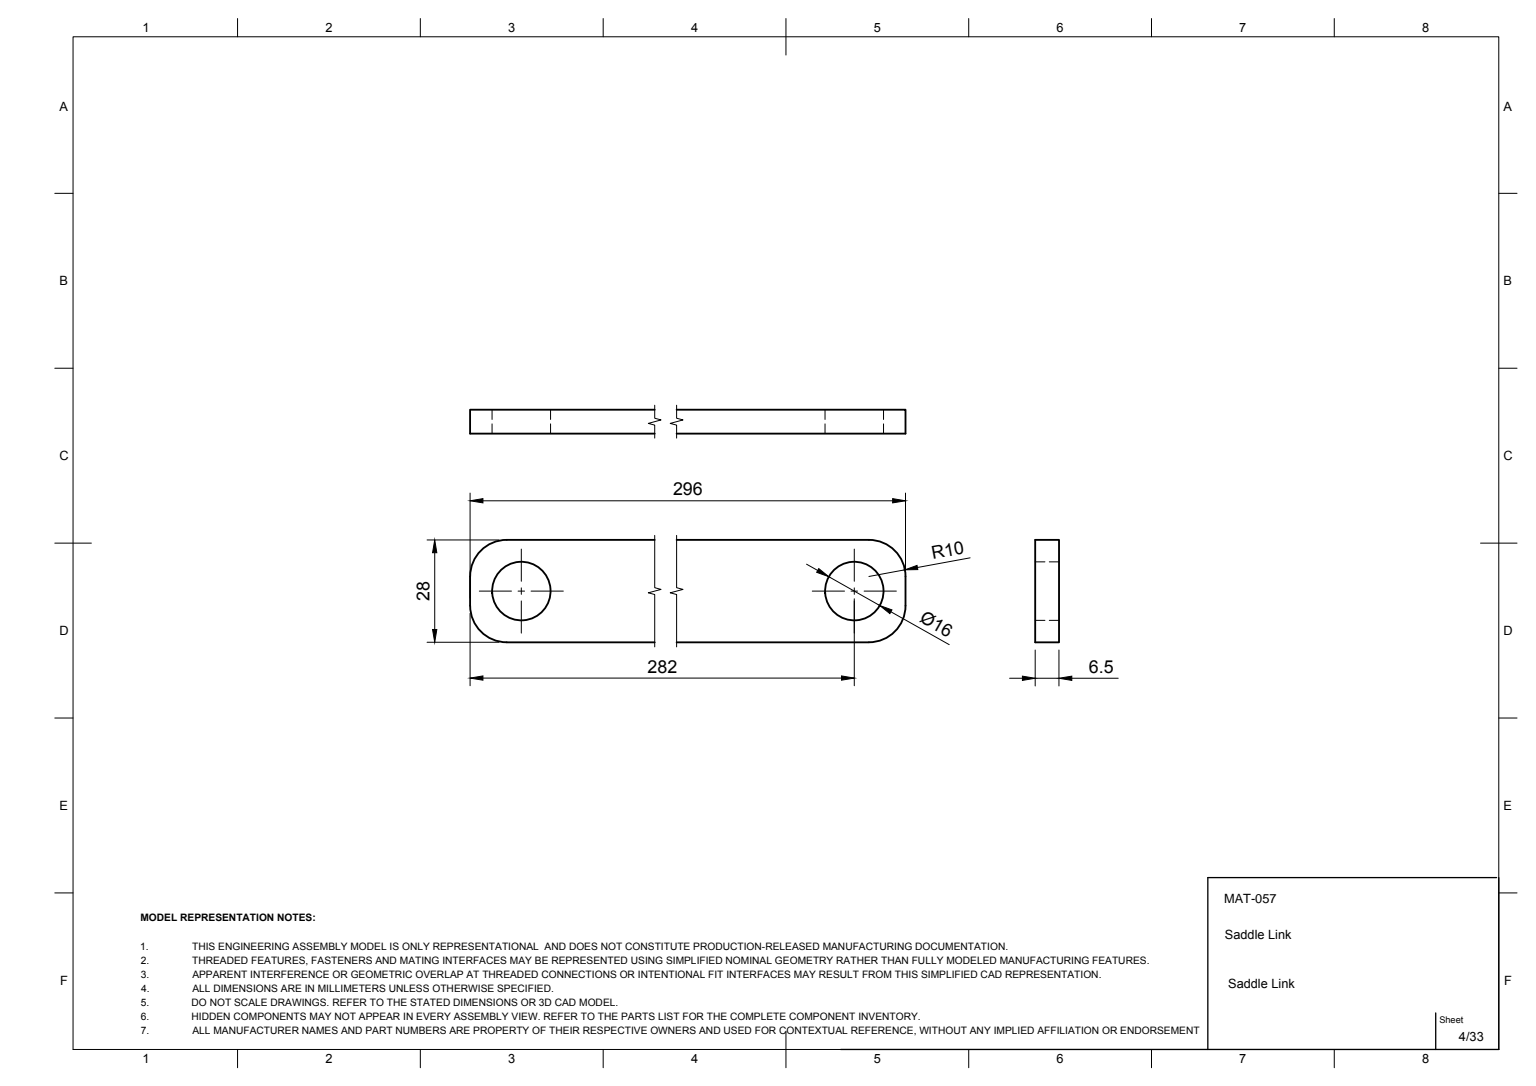
ISO-10303-21;
HEADER;
/* Generated by software containing ST-Developer
 * from STEP Tools, Inc. (www.steptools.com) 
 */

FILE_DESCRIPTION(
/* description */ ('STEP AP214', 'CAx-IF Rec.Pracs.---Representation and Presentation of Product Manufa
cturing Information (PMI)---4.0---2014-10-13'),
/* implementation_level */ '2;1');

FILE_NAME(
/* name */ 'Saddle Link.step',
/* time_stamp */ '2026-10-28T23:34:22+01:00',
/* author */ (''),
/* organization */ (''),
/* preprocessor_version */ 'ST-DEVELOPER v20.2',
/* originating_system */ 'Autodesk Translation Framework v15.17.0.0',
/* authorisation */ '');

FILE_SCHEMA (('AP242_MANAGED_MODEL_BASED_3D_ENGINEERING_MIM_LF { 1 0 10303 442 2 1 4 }'));
ENDSEC;

DATA;
#10=MECHANICAL_DESIGN_GEOMETRIC_PRESENTATION_REPRESENTATION('',(#258),#27807);
#212=SHAPE_REPRESENTATION_RELATIONSHIP('SRR','None',#27908,#234);
#234=ADVANCED_BREP_SHAPE_REPRESENTATION('',(#287),#27788);
#258=STYLED_ITEM('',(#28091),#287);
#287=MANIFOLD_SOLID_BREP('Body1',#12034);
#393=FACE_BOUND('',#2309,.T.);
#394=FACE_BOUND('',#2310,.T.);
#395=FACE_BOUND('',#2312,.T.);
#396=FACE_BOUND('',#2313,.T.);
#582=PLANE('',#12975);
#583=PLANE('',#12980);
#584=PLANE('',#12985);
#585=PLANE('',#12986);
#586=PLANE('',#12987);
#587=PLANE('',#12988);
#1093=CYLINDRICAL_SURFACE('',#12969,8.00000000000002);
#1094=CYLINDRICAL_SURFACE('',#12972,8.00000000000001);
#1095=CYLINDRICAL_SURFACE('',#12989,10.);
#1096=CYLINDRICAL_SURFACE('',#12990,9.99999999999999);
#1097=CYLINDRICAL_SURFACE('',#12991,10.);
#1098=CYLINDRICAL_SURFACE('',#12992,10.);
#1551=FACE_OUTER_BOUND('',#2306,.T.);
#1552=FACE_OUTER_BOUND('',#2307,.T.);
#1553=FACE_OUTER_BOUND('',#2308,.T.);
#1554=FACE_OUTER_BOUND('',#2311,.T.);
#1555=FACE_OUTER_BOUND('',#2314,.T.);
#1556=FACE_OUTER_BOUND('',#2315,.T.);
#1557=FACE_OUTER_BOUND('',#2316,.T.);
#1558=FACE_OUTER_BOUND('',#2317,.T.);
#1559=FACE_OUTER_BOUND('',#2318,.T.);
#1560=FACE_OUTER_BOUND('',#2319,.T.);
#1561=FACE_OUTER_BOUND('',#2320,.T.);
#1562=FACE_OUTER_BOUND('',#2321,.T.);
#2306=EDGE_LOOP('',(#9421,#9422,#9423,#9424));
#2307=EDGE_LOOP('',(#9425,#9426,#9427,#9428));
#2308=EDGE_LOOP('',(#9429,#9430,#9431,#9432,#9433,#9434,#9435,#9436));
#2309=EDGE_LOOP('',(#9437));
#2310=EDGE_LOOP('',(#9438));
#2311=EDGE_LOOP('',(#9439,#9440,#9441,#9442,#9443,#9444,#9445,#9446));
#2312=EDGE_LOOP('',(#9447));
#2313=EDGE_LOOP('',(#9448));
#2314=EDGE_LOOP('',(#9449,#9450,#9451,#9452));
#2315=EDGE_LOOP('',(#9453,#9454,#9455,#9456));
#2316=EDGE_LOOP('',(#9457,#9458,#9459,#9460));
#2317=EDGE_LOOP('',(#9461,#9462,#9463,#9464));
#2318=EDGE_LOOP('',(#9465,#9466,#9467,#9468));
#2319=EDGE_LOOP('',(#9469,#9470,#9471,#9472));
#2320=EDGE_LOOP('',(#9473,#9474,#9475,#9476));
#2321=EDGE_LOOP('',(#9477,#9478,#9479,#9480));
#3142=LINE('',#19340,#3962);
#3143=LINE('',#19346,#3963);
#3144=LINE('',#19351,#3964);
#3145=LINE('',#19355,#3965);
#3146=LINE('',#19359,#3966);
#3147=LINE('',#19363,#3967);
#3148=LINE('',#19368,#3968);
#3149=LINE('',#19372,#3969);
#3150=LINE('',#19376,#3970);
#3151=LINE('',#19380,#3971);
#3152=LINE('',#19383,#3972);
#3153=LINE('',#19384,#3973);
#3154=LINE('',#19386,#3974);
#3155=LINE('',#19387,#3975);
#3156=LINE('',#19389,#3976);
#3157=LINE('',#19390,#3977);
#3158=LINE('',#19392,#3978);
#3159=LINE('',#19393,#3979);
#3962=VECTOR('',#15466,8.00000000000002);
#3963=VECTOR('',#15473,8.00000000000001);
#3964=VECTOR('',#15478,1000.);
#3965=VECTOR('',#15481,1000.);
#3966=VECTOR('',#15484,1000.);
#3967=VECTOR('',#15487,1000.);
#3968=VECTOR('',#15492,1000.);
#3969=VECTOR('',#15495,1000.);
#3970=VECTOR('',#15498,1000.);
#3971=VECTOR('',#15501,1000.);
#3972=VECTOR('',#15506,1000.);
#3973=VECTOR('',#15507,1000.);
#3974=VECTOR('',#15510,1000.);
#3975=VECTOR('',#15511,1000.);
#3976=VECTOR('',#15514,1000.);
#3977=VECTOR('',#15515,1000.);
#3978=VECTOR('',#15518,1000.);
#3979=VECTOR('',#15519,1000.);
#4723=CIRCLE('',#12970,7.99999999999999);
#4724=CIRCLE('',#12971,7.99999999999999);
#4725=CIRCLE('',#12973,8.00000000000001);
#4726=CIRCLE('',#12974,8.00000000000001);
#4727=CIRCLE('',#12976,10.);
#4728=CIRCLE('',#12977,10.);
#4729=CIRCLE('',#12978,10.);
#4730=CIRCLE('',#12979,10.);
#4731=CIRCLE('',#12981,10.);
#4732=CIRCLE('',#12982,10.);
#4733=CIRCLE('',#12983,10.);
#4734=CIRCLE('',#12984,10.);
#5544=VERTEX_POINT('',#19337);
#5545=VERTEX_POINT('',#19339);
#5546=VERTEX_POINT('',#19343);
#5547=VERTEX_POINT('',#19345);
#5548=VERTEX_POINT('',#19349);
#5549=VERTEX_POINT('',#19350);
#5550=VERTEX_POINT('',#19352);
#5551=VERTEX_POINT('',#19354);
#5552=VERTEX_POINT('',#19356);
#5553=VERTEX_POINT('',#19358);
#5554=VERTEX_POINT('',#19360);
#5555=VERTEX_POINT('',#19362);
#5556=VERTEX_POINT('',#19366);
#5557=VERTEX_POINT('',#19367);
#5558=VERTEX_POINT('',#19369);
#5559=VERTEX_POINT('',#19371);
#5560=VERTEX_POINT('',#19373);
#5561=VERTEX_POINT('',#19375);
#5562=VERTEX_POINT('',#19377);
#5563=VERTEX_POINT('',#19379);
#6923=EDGE_CURVE('',#5544,#5544,#4723,.T.);
#6924=EDGE_CURVE('',#5544,#5545,#3142,.T.);
#6925=EDGE_CURVE('',#5545,#5545,#4724,.T.);
#6926=EDGE_CURVE('',#5546,#5546,#4725,.T.);
#6927=EDGE_CURVE('',#5546,#5547,#3143,.T.);
#6928=EDGE_CURVE('',#5547,#5547,#4726,.T.);
#6929=EDGE_CURVE('',#5548,#5549,#3144,.T.);
#6930=EDGE_CURVE('',#5549,#5550,#4727,.T.);
#6931=EDGE_CURVE('',#5550,#5551,#3145,.T.);
#6932=EDGE_CURVE('',#5551,#5552,#4728,.T.);
#6933=EDGE_CURVE('',#5552,#5553,#3146,.T.);
#6934=EDGE_CURVE('',#5553,#5554,#4729,.T.);
#6935=EDGE_CURVE('',#5554,#5555,#3147,.T.);
#6936=EDGE_CURVE('',#5555,#5548,#4730,.T.);
#6937=EDGE_CURVE('',#5556,#5557,#3148,.T.);
#6938=EDGE_CURVE('',#5556,#5558,#4731,.T.);
#6939=EDGE_CURVE('',#5559,#5558,#3149,.T.);
#6940=EDGE_CURVE('',#5559,#5560,#4732,.T.);
#6941=EDGE_CURVE('',#5561,#5560,#3150,.T.);
#6942=EDGE_CURVE('',#5561,#5562,#4733,.T.);
#6943=EDGE_CURVE('',#5563,#5562,#3151,.T.);
#6944=EDGE_CURVE('',#5563,#5557,#4734,.T.);
#6945=EDGE_CURVE('',#5550,#5556,#3152,.T.);
#6946=EDGE_CURVE('',#5557,#5551,#3153,.T.);
#6947=EDGE_CURVE('',#5552,#5563,#3154,.T.);
#6948=EDGE_CURVE('',#5562,#5553,#3155,.T.);
#6949=EDGE_CURVE('',#5560,#5555,#3156,.T.);
#6950=EDGE_CURVE('',#5554,#5561,#3157,.T.);
#6951=EDGE_CURVE('',#5558,#5549,#3158,.T.);
#6952=EDGE_CURVE('',#5548,#5559,#3159,.T.);
#9421=ORIENTED_EDGE('',*,*,#6923,.T.);
#9422=ORIENTED_EDGE('',*,*,#6924,.T.);
#9423=ORIENTED_EDGE('',*,*,#6925,.F.);
#9424=ORIENTED_EDGE('',*,*,#6924,.F.);
#9425=ORIENTED_EDGE('',*,*,#6926,.T.);
#9426=ORIENTED_EDGE('',*,*,#6927,.T.);
#9427=ORIENTED_EDGE('',*,*,#6928,.F.);
#9428=ORIENTED_EDGE('',*,*,#6927,.F.);
#9429=ORIENTED_EDGE('',*,*,#6929,.T.);
#9430=ORIENTED_EDGE('',*,*,#6930,.T.);
#9431=ORIENTED_EDGE('',*,*,#6931,.T.);
#9432=ORIENTED_EDGE('',*,*,#6932,.T.);
#9433=ORIENTED_EDGE('',*,*,#6933,.T.);
#9434=ORIENTED_EDGE('',*,*,#6934,.T.);
#9435=ORIENTED_EDGE('',*,*,#6935,.T.);
#9436=ORIENTED_EDGE('',*,*,#6936,.T.);
#9437=ORIENTED_EDGE('',*,*,#6923,.F.);
#9438=ORIENTED_EDGE('',*,*,#6926,.F.);
#9439=ORIENTED_EDGE('',*,*,#6937,.F.);
#9440=ORIENTED_EDGE('',*,*,#6938,.T.);
#9441=ORIENTED_EDGE('',*,*,#6939,.F.);
#9442=ORIENTED_EDGE('',*,*,#6940,.T.);
#9443=ORIENTED_EDGE('',*,*,#6941,.F.);
#9444=ORIENTED_EDGE('',*,*,#6942,.T.);
#9445=ORIENTED_EDGE('',*,*,#6943,.F.);
#9446=ORIENTED_EDGE('',*,*,#6944,.T.);
#9447=ORIENTED_EDGE('',*,*,#6928,.T.);
#9448=ORIENTED_EDGE('',*,*,#6925,.T.);
#9449=ORIENTED_EDGE('',*,*,#6931,.F.);
#9450=ORIENTED_EDGE('',*,*,#6945,.T.);
#9451=ORIENTED_EDGE('',*,*,#6937,.T.);
#9452=ORIENTED_EDGE('',*,*,#6946,.T.);
#9453=ORIENTED_EDGE('',*,*,#6933,.F.);
#9454=ORIENTED_EDGE('',*,*,#6947,.T.);
#9455=ORIENTED_EDGE('',*,*,#6943,.T.);
#9456=ORIENTED_EDGE('',*,*,#6948,.T.);
#9457=ORIENTED_EDGE('',*,*,#6941,.T.);
#9458=ORIENTED_EDGE('',*,*,#6949,.T.);
#9459=ORIENTED_EDGE('',*,*,#6935,.F.);
#9460=ORIENTED_EDGE('',*,*,#6950,.T.);
#9461=ORIENTED_EDGE('',*,*,#6939,.T.);
#9462=ORIENTED_EDGE('',*,*,#6951,.T.);
#9463=ORIENTED_EDGE('',*,*,#6929,.F.);
#9464=ORIENTED_EDGE('',*,*,#6952,.T.);
#9465=ORIENTED_EDGE('',*,*,#6930,.F.);
#9466=ORIENTED_EDGE('',*,*,#6951,.F.);
#9467=ORIENTED_EDGE('',*,*,#6938,.F.);
#9468=ORIENTED_EDGE('',*,*,#6945,.F.);
#9469=ORIENTED_EDGE('',*,*,#6932,.F.);
#9470=ORIENTED_EDGE('',*,*,#6946,.F.);
#9471=ORIENTED_EDGE('',*,*,#6944,.F.);
#9472=ORIENTED_EDGE('',*,*,#6947,.F.);
#9473=ORIENTED_EDGE('',*,*,#6936,.F.);
#9474=ORIENTED_EDGE('',*,*,#6949,.F.);
#9475=ORIENTED_EDGE('',*,*,#6940,.F.);
#9476=ORIENTED_EDGE('',*,*,#6952,.F.);
#9477=ORIENTED_EDGE('',*,*,#6934,.F.);
#9478=ORIENTED_EDGE('',*,*,#6948,.F.);
#9479=ORIENTED_EDGE('',*,*,#6942,.F.);
#9480=ORIENTED_EDGE('',*,*,#6950,.F.);
#11633=ADVANCED_FACE('',(#1551),#1093,.F.);
#11634=ADVANCED_FACE('',(#1552),#1094,.F.);
#11635=ADVANCED_FACE('',(#1553,#393,#394),#582,.T.);
#11636=ADVANCED_FACE('',(#1554,#395,#396),#583,.F.);
#11637=ADVANCED_FACE('',(#1555),#584,.F.);
#11638=ADVANCED_FACE('',(#1556),#585,.F.);
#11639=ADVANCED_FACE('',(#1557),#586,.F.);
#11640=ADVANCED_FACE('',(#1558),#587,.F.);
#11641=ADVANCED_FACE('',(#1559),#1095,.T.);
#11642=ADVANCED_FACE('',(#1560),#1096,.T.);
#11643=ADVANCED_FACE('',(#1561),#1097,.T.);
#11644=ADVANCED_FACE('',(#1562),#1098,.T.);
#12034=CLOSED_SHELL('',(#11633,#11634,#11635,#11636,#11637,#11638,#11639,
#11640,#11641,#11642,#11643,#11644));
#12968=AXIS2_PLACEMENT_3D('',#19335,#15460,#15461);
#12969=AXIS2_PLACEMENT_3D('',#19336,#15462,#15463);
#12970=AXIS2_PLACEMENT_3D('',#19338,#15464,#15465);
#12971=AXIS2_PLACEMENT_3D('',#19341,#15467,#15468);
#12972=AXIS2_PLACEMENT_3D('',#19342,#15469,#15470);
#12973=AXIS2_PLACEMENT_3D('',#19344,#15471,#15472);
#12974=AXIS2_PLACEMENT_3D('',#19347,#15474,#15475);
#12975=AXIS2_PLACEMENT_3D('',#19348,#15476,#15477);
#12976=AXIS2_PLACEMENT_3D('',#19353,#15479,#15480);
#12977=AXIS2_PLACEMENT_3D('',#19357,#15482,#15483);
#12978=AXIS2_PLACEMENT_3D('',#19361,#15485,#15486);
#12979=AXIS2_PLACEMENT_3D('',#19364,#15488,#15489);
#12980=AXIS2_PLACEMENT_3D('',#19365,#15490,#15491);
#12981=AXIS2_PLACEMENT_3D('',#19370,#15493,#15494);
#12982=AXIS2_PLACEMENT_3D('',#19374,#15496,#15497);
#12983=AXIS2_PLACEMENT_3D('',#19378,#15499,#15500);
#12984=AXIS2_PLACEMENT_3D('',#19381,#15502,#15503);
#12985=AXIS2_PLACEMENT_3D('',#19382,#15504,#15505);
#12986=AXIS2_PLACEMENT_3D('',#19385,#15508,#15509);
#12987=AXIS2_PLACEMENT_3D('',#19388,#15512,#15513);
#12988=AXIS2_PLACEMENT_3D('',#19391,#15516,#15517);
#12989=AXIS2_PLACEMENT_3D('',#19394,#15520,#15521);
#12990=AXIS2_PLACEMENT_3D('',#19395,#15522,#15523);
#12991=AXIS2_PLACEMENT_3D('',#19396,#15524,#15525);
#12992=AXIS2_PLACEMENT_3D('',#19397,#15526,#15527);
#15460=DIRECTION('axis',(0.,0.,1.));
#15461=DIRECTION('refdir',(1.,0.,0.));
#15462=DIRECTION('center_axis',(1.34374111916937E-16,-6.5016645363134E-17,
1.));
#15463=DIRECTION('ref_axis',(0.997400584683992,-0.0720560453538152,-1.38709660139384E-16));
#15464=DIRECTION('center_axis',(-1.34374111916937E-16,6.5016645363134E-17,
-1.));
#15465=DIRECTION('ref_axis',(-0.997400584683992,0.0720560453538154,1.38709660139384E-16));
#15466=DIRECTION('',(1.34374111916937E-16,-6.5016645363134E-17,1.));
#15467=DIRECTION('center_axis',(-1.34374111916937E-16,6.5016645363134E-17,
-1.));
#15468=DIRECTION('ref_axis',(-0.997400584683992,0.0720560453538154,1.38709660139384E-16));
#15469=DIRECTION('center_axis',(1.34374111916937E-16,-6.5016645363134E-17,
1.));
#15470=DIRECTION('ref_axis',(0.997400584683992,-0.0720560453538153,-1.38709660139384E-16));
#15471=DIRECTION('center_axis',(-1.34374111916937E-16,6.5016645363134E-17,
-1.));
#15472=DIRECTION('ref_axis',(-0.997400584683992,0.0720560453538153,1.38709660139384E-16));
#15473=DIRECTION('',(1.34374111916937E-16,-6.5016645363134E-17,1.));
#15474=DIRECTION('center_axis',(-1.34374111916937E-16,6.5016645363134E-17,
-1.));
#15475=DIRECTION('ref_axis',(-0.997400584683992,0.0720560453538153,1.38709660139384E-16));
#15476=DIRECTION('center_axis',(-9.47320768979473E-17,6.21527526432887E-17,
-1.));
#15477=DIRECTION('ref_axis',(-0.997400584683992,0.072056045353816,9.89643104496708E-17));
#15478=DIRECTION('',(-0.997400584683992,0.072056045353816,9.89643104496708E-17));
#15479=DIRECTION('center_axis',(-1.34374111916937E-16,6.5016645363134E-17,
-1.));
#15480=DIRECTION('ref_axis',(-0.997400584683992,0.0720560453538159,1.38709660139384E-16));
#15481=DIRECTION('',(0.0720560453538158,0.997400584683992,6.43240143985008E-17));
#15482=DIRECTION('center_axis',(-1.34374111916937E-16,6.5016645363134E-17,
-1.));
#15483=DIRECTION('ref_axis',(-0.997400584683992,0.0720560453538159,1.38709660139384E-16));
#15484=DIRECTION('',(0.997400584683992,-0.072056045353816,-9.89643104496708E-17));
#15485=DIRECTION('center_axis',(-1.34374111916937E-16,6.5016645363134E-17,
-1.));
#15486=DIRECTION('ref_axis',(-0.997400584683992,0.072056045353816,1.38709660139384E-16));
#15487=DIRECTION('',(-0.0720560453538158,-0.997400584683992,-6.43240143985008E-17));
#15488=DIRECTION('center_axis',(-1.34374111916937E-16,6.5016645363134E-17,
-1.));
#15489=DIRECTION('ref_axis',(-0.997400584683992,0.072056045353816,1.38709660139384E-16));
#15490=DIRECTION('center_axis',(-9.47320768979473E-17,6.21527526432887E-17,
-1.));
#15491=DIRECTION('ref_axis',(-0.997400584683992,0.072056045353816,9.89643104496708E-17));
#15492=DIRECTION('',(0.0720560453538158,0.997400584683992,6.43240143985008E-17));
#15493=DIRECTION('center_axis',(1.34374111916937E-16,-6.5016645363134E-17,
1.));
#15494=DIRECTION('ref_axis',(-0.997400584683992,0.0720560453538159,1.38709660139384E-16));
#15495=DIRECTION('',(-0.997400584683992,0.072056045353816,9.89643104496708E-17));
#15496=DIRECTION('center_axis',(1.34374111916937E-16,-6.5016645363134E-17,
1.));
#15497=DIRECTION('ref_axis',(-0.997400584683992,0.0720560453538174,1.38709660139384E-16));
#15498=DIRECTION('',(-0.0720560453538158,-0.997400584683992,-6.43240143985008E-17));
#15499=DIRECTION('center_axis',(1.34374111916937E-16,-6.5016645363134E-17,
1.));
#15500=DIRECTION('ref_axis',(-0.997400584683992,0.072056045353816,1.38709660139384E-16));
#15501=DIRECTION('',(0.997400584683992,-0.072056045353816,-9.89643104496708E-17));
#15502=DIRECTION('center_axis',(1.34374111916937E-16,-6.5016645363134E-17,
1.));
#15503=DIRECTION('ref_axis',(-0.997400584683992,0.0720560453538076,1.38709660139383E-16));
#15504=DIRECTION('center_axis',(0.997400584683992,-0.0720560453538159,-1.38709660139384E-16));
#15505=DIRECTION('ref_axis',(-1.34374111916937E-16,6.5016645363134E-17,
-1.));
#15506=DIRECTION('',(1.34374111916937E-16,-6.5016645363134E-17,1.));
#15507=DIRECTION('',(-1.34374111916937E-16,6.5016645363134E-17,-1.));
#15508=DIRECTION('center_axis',(-0.0720560453538158,-0.997400584683992,
-5.51651729967161E-17));
#15509=DIRECTION('ref_axis',(1.34374111916937E-16,-6.5016645363134E-17,
1.));
#15510=DIRECTION('',(1.34374111916937E-16,-6.5016645363134E-17,1.));
#15511=DIRECTION('',(-1.34374111916937E-16,6.5016645363134E-17,-1.));
#15512=DIRECTION('center_axis',(-0.997400584683992,0.0720560453538159,1.38709660139384E-16));
#15513=DIRECTION('ref_axis',(1.34374111916937E-16,-6.5016645363134E-17,
1.));
#15514=DIRECTION('',(-1.34374111916937E-16,6.5016645363134E-17,-1.));
#15515=DIRECTION('',(1.34374111916937E-16,-6.5016645363134E-17,1.));
#15516=DIRECTION('center_axis',(0.0720560453538158,0.997400584683992,5.51651729967161E-17));
#15517=DIRECTION('ref_axis',(-1.34374111916937E-16,6.5016645363134E-17,
-1.));
#15518=DIRECTION('',(-1.34374111916937E-16,6.5016645363134E-17,-1.));
#15519=DIRECTION('',(1.34374111916937E-16,-6.5016645363134E-17,1.));
#15520=DIRECTION('center_axis',(1.34374111916937E-16,-6.5016645363134E-17,
1.));
#15521=DIRECTION('ref_axis',(0.997400584683992,-0.0720560453538159,-1.38709660139384E-16));
#15522=DIRECTION('center_axis',(1.34374111916937E-16,-6.5016645363134E-17,
1.));
#15523=DIRECTION('ref_axis',(0.997400584683992,-0.0720560453538161,-1.38709660139384E-16));
#15524=DIRECTION('center_axis',(1.34374111916937E-16,-6.5016645363134E-17,
1.));
#15525=DIRECTION('ref_axis',(0.997400584683992,-0.072056045353816,-1.38709660139384E-16));
#15526=DIRECTION('center_axis',(1.34374111916937E-16,-6.5016645363134E-17,
1.));
#15527=DIRECTION('ref_axis',(0.997400584683992,-0.072056045353816,-1.38709660139384E-16));
#19335=CARTESIAN_POINT('',(0.,0.,0.));
#19336=CARTESIAN_POINT('Origin',(-256.262104047423,132.050757761858,278.073593133703));
#19337=CARTESIAN_POINT('',(-264.241308724895,132.627206124688,278.073593133703));
#19338=CARTESIAN_POINT('Origin',(-256.262104047423,132.050757761858,278.073593133703));
#19339=CARTESIAN_POINT('',(-264.241308724895,132.627206124688,284.573593133703));
#19340=CARTESIAN_POINT('',(-264.241308724895,132.627206124688,278.073593133703));
#19341=CARTESIAN_POINT('Origin',(-256.262104047423,132.050757761858,284.573593133703));
#19342=CARTESIAN_POINT('Origin',(11.0412526478865,112.739737607035,278.073593133703));
#19343=CARTESIAN_POINT('',(3.06204797041458,113.316185969866,278.073593133703));
#19344=CARTESIAN_POINT('Origin',(11.0412526478865,112.739737607035,278.073593133703));
#19345=CARTESIAN_POINT('',(3.06204797041458,113.316185969866,284.573593133703));
#19346=CARTESIAN_POINT('',(3.06204797041458,113.316185969866,278.073593133703));
#19347=CARTESIAN_POINT('Origin',(11.0412526478865,112.739737607035,284.573593133703));
#19348=CARTESIAN_POINT('Origin',(-122.610425699768,122.395247684447,278.073593133703));
#19349=CARTESIAN_POINT('',(14.022070351669,98.487905240044,278.073593133703));
#19350=CARTESIAN_POINT('',(-261.260491021113,118.375373757697,278.073593133703));
#19351=CARTESIAN_POINT('',(23.9960761985089,97.7673447865059,278.073593133703));
#19352=CARTESIAN_POINT('',(-270.513936414414,129.069940058075,278.073593133703));
#19353=CARTESIAN_POINT('Origin',(-260.539930567575,128.349379604537,278.073593133703));
#19354=CARTESIAN_POINT('',(-269.937488051584,137.049144735547,278.073593133703));
#19355=CARTESIAN_POINT('',(-269.216927598046,147.023150582387,278.073593133703));
#19356=CARTESIAN_POINT('',(-259.242921751206,146.302590128849,278.073593133703));
#19357=CARTESIAN_POINT('Origin',(-259.963482204744,136.328584282009,278.073593133703));
#19358=CARTESIAN_POINT('',(16.0396396215758,126.415121611196,278.073593133703));
#19359=CARTESIAN_POINT('',(26.0136454684158,125.694561157658,278.073593133703));
#19360=CARTESIAN_POINT('',(25.2930850148776,115.720555310818,278.073593133703));
#19361=CARTESIAN_POINT('Origin',(15.3190791680377,116.441115764356,278.073593133703));
#19362=CARTESIAN_POINT('',(24.7166366520471,107.741350633346,278.073593133703));
#19363=CARTESIAN_POINT('',(26.0136454684158,125.694561157658,278.073593133703));
#19364=CARTESIAN_POINT('Origin',(14.7426308052072,108.461911086884,278.073593133703));
#19365=CARTESIAN_POINT('Origin',(-122.610425699768,122.395247684447,284.573593133703));
#19366=CARTESIAN_POINT('',(-270.513936414414,129.069940058075,284.573593133703));
#19367=CARTESIAN_POINT('',(-269.937488051584,137.049144735547,284.573593133703));
#19368=CARTESIAN_POINT('',(-269.216927598046,147.023150582387,284.573593133703));
#19369=CARTESIAN_POINT('',(-261.260491021113,118.375373757697,284.573593133703));
#19370=CARTESIAN_POINT('Origin',(-260.539930567575,128.349379604537,284.573593133703));
#19371=CARTESIAN_POINT('',(14.022070351669,98.487905240044,284.573593133703));
#19372=CARTESIAN_POINT('',(23.9960761985089,97.7673447865059,284.573593133703));
#19373=CARTESIAN_POINT('',(24.7166366520471,107.741350633346,284.573593133703));
#19374=CARTESIAN_POINT('Origin',(14.7426308052072,108.461911086884,284.573593133703));
#19375=CARTESIAN_POINT('',(25.2930850148776,115.720555310818,284.573593133703));
#19376=CARTESIAN_POINT('',(26.0136454684158,125.694561157658,284.573593133703));
#19377=CARTESIAN_POINT('',(16.0396396215758,126.415121611196,284.573593133703));
#19378=CARTESIAN_POINT('Origin',(15.3190791680377,116.441115764356,284.573593133703));
#19379=CARTESIAN_POINT('',(-259.242921751206,146.302590128849,284.573593133703));
#19380=CARTESIAN_POINT('',(26.0136454684158,125.694561157658,284.573593133703));
#19381=CARTESIAN_POINT('Origin',(-259.963482204744,136.328584282009,284.573593133703));
#19382=CARTESIAN_POINT('Origin',(-269.216927598046,147.023150582387,278.073593133703));
#19383=CARTESIAN_POINT('',(-270.513936414414,129.069940058075,278.073593133703));
#19384=CARTESIAN_POINT('',(-269.937488051584,137.049144735547,278.073593133703));
#19385=CARTESIAN_POINT('Origin',(26.0136454684158,125.694561157658,278.073593133703));
#19386=CARTESIAN_POINT('',(-259.242921751206,146.302590128849,278.073593133703));
#19387=CARTESIAN_POINT('',(16.0396396215758,126.415121611196,278.073593133703));
#19388=CARTESIAN_POINT('Origin',(26.0136454684158,125.694561157658,278.073593133703));
#19389=CARTESIAN_POINT('',(24.7166366520471,107.741350633346,278.073593133703));
#19390=CARTESIAN_POINT('',(25.2930850148776,115.720555310818,278.073593133703));
#19391=CARTESIAN_POINT('Origin',(23.9960761985089,97.7673447865059,278.073593133703));
#19392=CARTESIAN_POINT('',(-261.260491021113,118.375373757697,278.073593133703));
#19393=CARTESIAN_POINT('',(14.022070351669,98.487905240044,278.073593133703));
#19394=CARTESIAN_POINT('Origin',(-260.539930567575,128.349379604537,278.073593133703));
#19395=CARTESIAN_POINT('Origin',(-259.963482204744,136.328584282009,278.073593133703));
#19396=CARTESIAN_POINT('Origin',(14.7426308052072,108.461911086884,278.073593133703));
#19397=CARTESIAN_POINT('Origin',(15.3190791680377,116.441115764356,278.073593133703));
#27759=UNCERTAINTY_MEASURE_WITH_UNIT(LENGTH_MEASURE(0.01),#27808,
'DISTANCE_ACCURACY_VALUE',
'Maximum model space distance between geometric entities at asserted c
onnectivities');
#27778=UNCERTAINTY_MEASURE_WITH_UNIT(LENGTH_MEASURE(0.01),#27808,
'DISTANCE_ACCURACY_VALUE',
'Maximum model space distance between geometric entities at asserted c
onnectivities');
#27788=(
GEOMETRIC_REPRESENTATION_CONTEXT(3)
GLOBAL_UNCERTAINTY_ASSIGNED_CONTEXT((#27759))
GLOBAL_UNIT_ASSIGNED_CONTEXT((#27808,#27810,#27811))
REPRESENTATION_CONTEXT('','3D')
);
#27807=(
GEOMETRIC_REPRESENTATION_CONTEXT(3)
GLOBAL_UNCERTAINTY_ASSIGNED_CONTEXT((#27778))
GLOBAL_UNIT_ASSIGNED_CONTEXT((#27808,#27810,#27811))
REPRESENTATION_CONTEXT('','3D')
);
#27808=(
LENGTH_UNIT()
NAMED_UNIT(*)
SI_UNIT(.MILLI.,.METRE.)
);
#27810=(
NAMED_UNIT(*)
PLANE_ANGLE_UNIT()
SI_UNIT($,.RADIAN.)
);
#27811=(
NAMED_UNIT(*)
SI_UNIT($,.STERADIAN.)
SOLID_ANGLE_UNIT()
);
#27821=SHAPE_DEFINITION_REPRESENTATION(#27854,#27908);
#27854=PRODUCT_DEFINITION_SHAPE('',$,#27937);
#27908=SHAPE_REPRESENTATION('',(#12968),#27788);
#27927=PRODUCT_DEFINITION_CONTEXT('part definition',#28013,'design');
#27937=PRODUCT_DEFINITION('Saddle Link','Saddle Link',#27965,#27927);
#27965=PRODUCT_DEFINITION_FORMATION('',$,#28024);
#28013=APPLICATION_CONTEXT('Managed model based 3d engineering');
#28014=PRODUCT_CONTEXT('part definition',#28013,'mechanical');
#28024=PRODUCT('Saddle Link','Saddle Link',$,(#28014));
#28085=COLOUR_RGB('Off White',0.89,0.88,0.83);
#28086=FILL_AREA_STYLE_COLOUR('',#28085);
#28087=FILL_AREA_STYLE('',(#28086));
#28088=SURFACE_STYLE_FILL_AREA(#28087);
#28089=SURFACE_SIDE_STYLE('',(#28088));
#28090=SURFACE_STYLE_USAGE(.BOTH.,#28089);
#28091=PRESENTATION_STYLE_ASSIGNMENT((#28090));
ENDSEC;
END-ISO-10303-21;
